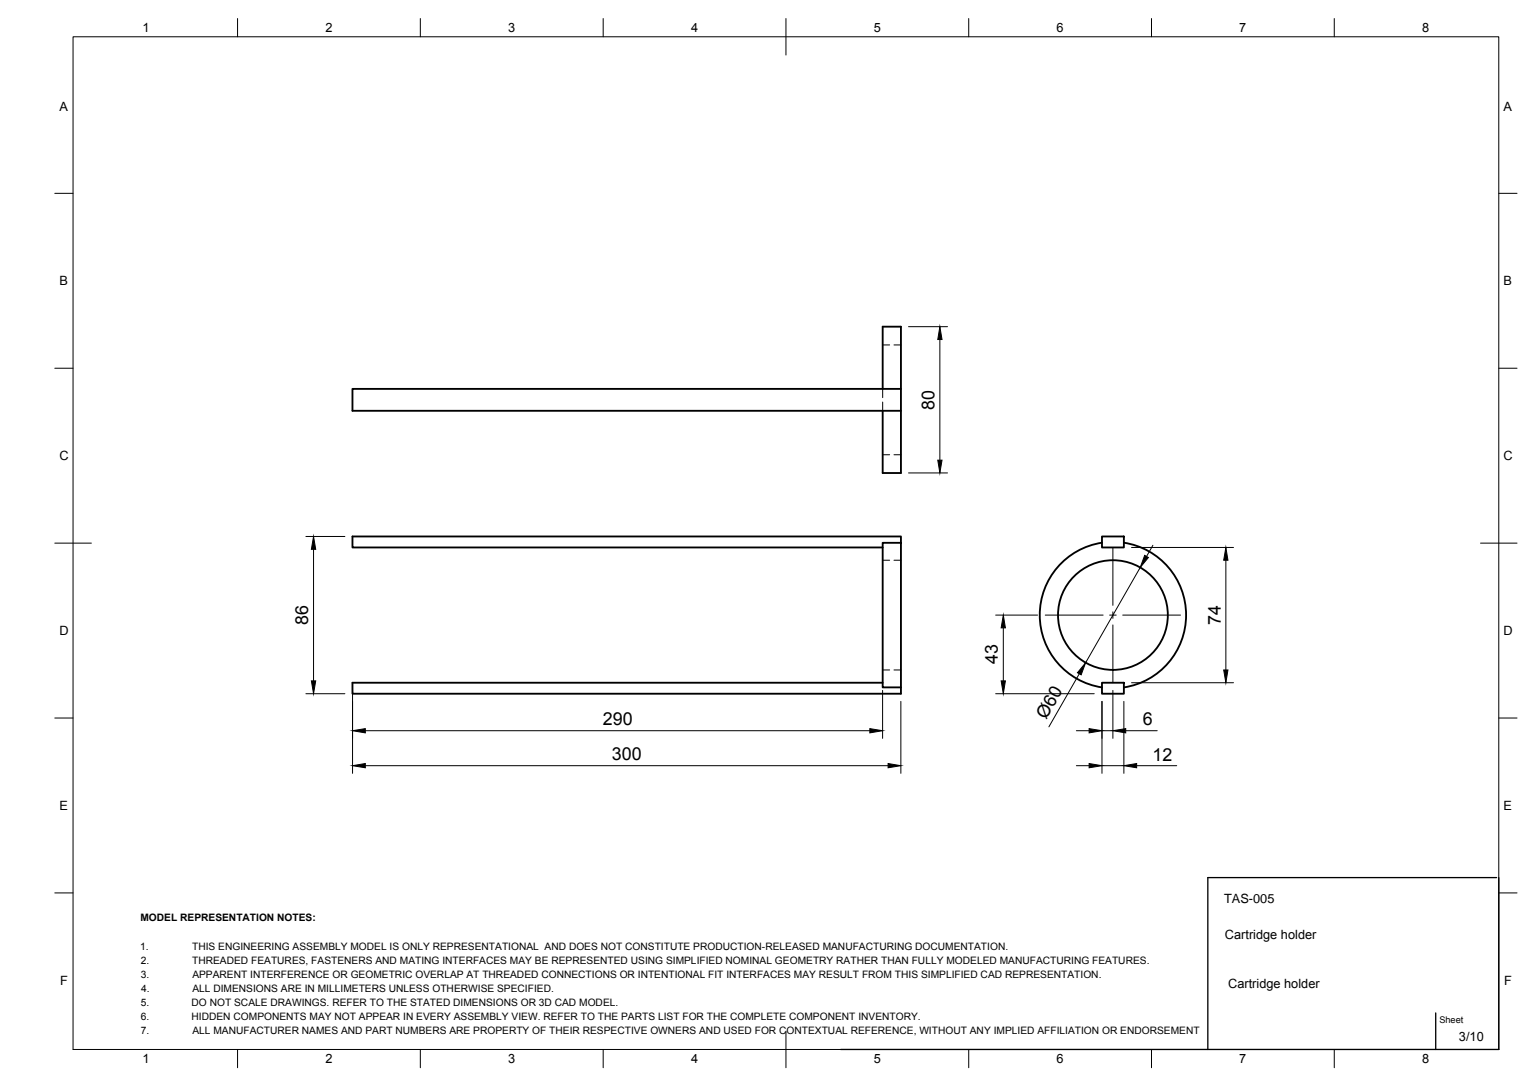
ISO-10303-21;
HEADER;
/* Generated by software containing ST-Developer
 * from STEP Tools, Inc. (www.steptools.com) 
 */

FILE_DESCRIPTION(
/* description */ ('STEP AP214'),
/* implementation_level */ '2;1');

FILE_NAME(
/* name */ 'Cartridge holder.step',
/* time_stamp */ '2026-11-04T19:54:22-08:00',
/* author */ (''),
/* organization */ (''),
/* preprocessor_version */ 'ST-DEVELOPER v20.2',
/* originating_system */ 'Autodesk Translation Framework v15.17.0.0',
/* authorisation */ '');

FILE_SCHEMA (('AUTOMOTIVE_DESIGN { 1 0 10303 214 3 1 1 }'));
ENDSEC;

DATA;
#10=MECHANICAL_DESIGN_GEOMETRIC_PRESENTATION_REPRESENTATION('',(#239),#14084);
#221=SHAPE_REPRESENTATION_RELATIONSHIP('SRR','None',#14120,#230);
#230=ADVANCED_BREP_SHAPE_REPRESENTATION('',(#248),#14075);
#239=STYLED_ITEM('',(#14174),#248);
#248=MANIFOLD_SOLID_BREP('Body1',#3465);
#257=FACE_BOUND('',#558,.T.);
#258=FACE_BOUND('',#561,.T.);
#285=PLANE('',#3582);
#286=PLANE('',#3586);
#287=PLANE('',#3587);
#288=PLANE('',#3588);
#289=PLANE('',#3589);
#290=PLANE('',#3590);
#291=PLANE('',#3591);
#292=PLANE('',#3592);
#293=PLANE('',#3593);
#294=PLANE('',#3594);
#295=PLANE('',#3595);
#296=PLANE('',#3596);
#365=FACE_OUTER_BOUND('',#555,.T.);
#366=FACE_OUTER_BOUND('',#556,.T.);
#367=FACE_OUTER_BOUND('',#557,.T.);
#368=FACE_OUTER_BOUND('',#559,.T.);
#369=FACE_OUTER_BOUND('',#560,.T.);
#370=FACE_OUTER_BOUND('',#562,.T.);
#371=FACE_OUTER_BOUND('',#563,.T.);
#372=FACE_OUTER_BOUND('',#564,.T.);
#373=FACE_OUTER_BOUND('',#565,.T.);
#374=FACE_OUTER_BOUND('',#566,.T.);
#375=FACE_OUTER_BOUND('',#567,.T.);
#376=FACE_OUTER_BOUND('',#568,.T.);
#377=FACE_OUTER_BOUND('',#569,.T.);
#378=FACE_OUTER_BOUND('',#570,.T.);
#379=FACE_OUTER_BOUND('',#571,.T.);
#555=EDGE_LOOP('',(#2197,#2198,#2199,#2200));
#556=EDGE_LOOP('',(#2201,#2202,#2203,#2204));
#557=EDGE_LOOP('',(#2205,#2206,#2207,#2208,#2209,#2210,#2211,#2212));
#558=EDGE_LOOP('',(#2213));
#559=EDGE_LOOP('',(#2214,#2215,#2216,#2217));
#560=EDGE_LOOP('',(#2218,#2219,#2220,#2221,#2222,#2223,#2224,#2225));
#561=EDGE_LOOP('',(#2226));
#562=EDGE_LOOP('',(#2227,#2228,#2229,#2230));
#563=EDGE_LOOP('',(#2231,#2232,#2233,#2234,#2235,#2236));
#564=EDGE_LOOP('',(#2237,#2238,#2239,#2240));
#565=EDGE_LOOP('',(#2241,#2242,#2243,#2244,#2245,#2246));
#566=EDGE_LOOP('',(#2247,#2248,#2249,#2250));
#567=EDGE_LOOP('',(#2251,#2252,#2253,#2254));
#568=EDGE_LOOP('',(#2255,#2256,#2257,#2258,#2259,#2260));
#569=EDGE_LOOP('',(#2261,#2262,#2263,#2264));
#570=EDGE_LOOP('',(#2265,#2266,#2267,#2268,#2269,#2270));
#571=EDGE_LOOP('',(#2271,#2272,#2273,#2274));
#773=LINE('',#4707,#1030);
#774=LINE('',#4714,#1031);
#775=LINE('',#4717,#1032);
#776=LINE('',#4720,#1033);
#777=LINE('',#4722,#1034);
#778=LINE('',#4724,#1035);
#779=LINE('',#4728,#1036);
#780=LINE('',#4730,#1037);
#781=LINE('',#4731,#1038);
#782=LINE('',#4734,#1039);
#783=LINE('',#4737,#1040);
#784=LINE('',#4740,#1041);
#785=LINE('',#4742,#1042);
#786=LINE('',#4743,#1043);
#787=LINE('',#4745,#1044);
#788=LINE('',#4747,#1045);
#789=LINE('',#4748,#1046);
#790=LINE('',#4751,#1047);
#791=LINE('',#4753,#1048);
#792=LINE('',#4754,#1049);
#793=LINE('',#4757,#1050);
#794=LINE('',#4758,#1051);
#795=LINE('',#4761,#1052);
#796=LINE('',#4762,#1053);
#797=LINE('',#4764,#1054);
#798=LINE('',#4768,#1055);
#799=LINE('',#4770,#1056);
#800=LINE('',#4771,#1057);
#801=LINE('',#4774,#1058);
#802=LINE('',#4775,#1059);
#803=LINE('',#4778,#1060);
#804=LINE('',#4779,#1061);
#805=LINE('',#4781,#1062);
#1030=VECTOR('',#3872,30.);
#1031=VECTOR('',#3879,1000.);
#1032=VECTOR('',#3882,1000.);
#1033=VECTOR('',#3885,1000.);
#1034=VECTOR('',#3886,1000.);
#1035=VECTOR('',#3887,1000.);
#1036=VECTOR('',#3890,1000.);
#1037=VECTOR('',#3891,1000.);
#1038=VECTOR('',#3892,1000.);
#1039=VECTOR('',#3895,1000.);
#1040=VECTOR('',#3898,1000.);
#1041=VECTOR('',#3901,1000.);
#1042=VECTOR('',#3902,1000.);
#1043=VECTOR('',#3903,1000.);
#1044=VECTOR('',#3904,1000.);
#1045=VECTOR('',#3905,1000.);
#1046=VECTOR('',#3906,1000.);
#1047=VECTOR('',#3909,1000.);
#1048=VECTOR('',#3910,1000.);
#1049=VECTOR('',#3911,1000.);
#1050=VECTOR('',#3914,1000.);
#1051=VECTOR('',#3915,1000.);
#1052=VECTOR('',#3918,1000.);
#1053=VECTOR('',#3919,1000.);
#1054=VECTOR('',#3922,1000.);
#1055=VECTOR('',#3927,1000.);
#1056=VECTOR('',#3928,1000.);
#1057=VECTOR('',#3929,1000.);
#1058=VECTOR('',#3932,1000.);
#1059=VECTOR('',#3933,1000.);
#1060=VECTOR('',#3936,1000.);
#1061=VECTOR('',#3937,1000.);
#1062=VECTOR('',#3940,1000.);
#1287=CIRCLE('',#3577,30.);
#1288=CIRCLE('',#3578,30.);
#1289=CIRCLE('',#3580,40.);
#1290=CIRCLE('',#3581,40.);
#1291=CIRCLE('',#3583,40.);
#1292=CIRCLE('',#3585,40.);
#1377=VERTEX_POINT('',#4704);
#1378=VERTEX_POINT('',#4706);
#1379=VERTEX_POINT('',#4710);
#1380=VERTEX_POINT('',#4711);
#1381=VERTEX_POINT('',#4713);
#1382=VERTEX_POINT('',#4715);
#1383=VERTEX_POINT('',#4719);
#1384=VERTEX_POINT('',#4721);
#1385=VERTEX_POINT('',#4723);
#1386=VERTEX_POINT('',#4725);
#1387=VERTEX_POINT('',#4727);
#1388=VERTEX_POINT('',#4729);
#1389=VERTEX_POINT('',#4733);
#1390=VERTEX_POINT('',#4735);
#1391=VERTEX_POINT('',#4739);
#1392=VERTEX_POINT('',#4741);
#1393=VERTEX_POINT('',#4744);
#1394=VERTEX_POINT('',#4746);
#1395=VERTEX_POINT('',#4750);
#1396=VERTEX_POINT('',#4752);
#1397=VERTEX_POINT('',#4756);
#1398=VERTEX_POINT('',#4760);
#1399=VERTEX_POINT('',#4767);
#1400=VERTEX_POINT('',#4769);
#1401=VERTEX_POINT('',#4773);
#1402=VERTEX_POINT('',#4777);
#1702=EDGE_CURVE('',#1377,#1377,#1287,.T.);
#1703=EDGE_CURVE('',#1377,#1378,#773,.T.);
#1704=EDGE_CURVE('',#1378,#1378,#1288,.T.);
#1705=EDGE_CURVE('',#1379,#1380,#1289,.T.);
#1706=EDGE_CURVE('',#1381,#1379,#774,.T.);
#1707=EDGE_CURVE('',#1381,#1382,#1290,.T.);
#1708=EDGE_CURVE('',#1380,#1382,#775,.T.);
#1709=EDGE_CURVE('',#1380,#1383,#776,.T.);
#1710=EDGE_CURVE('',#1383,#1384,#777,.T.);
#1711=EDGE_CURVE('',#1384,#1385,#778,.T.);
#1712=EDGE_CURVE('',#1385,#1386,#1291,.T.);
#1713=EDGE_CURVE('',#1386,#1387,#779,.T.);
#1714=EDGE_CURVE('',#1387,#1388,#780,.T.);
#1715=EDGE_CURVE('',#1388,#1379,#781,.T.);
#1716=EDGE_CURVE('',#1389,#1385,#782,.T.);
#1717=EDGE_CURVE('',#1389,#1390,#1292,.T.);
#1718=EDGE_CURVE('',#1386,#1390,#783,.T.);
#1719=EDGE_CURVE('',#1391,#1389,#784,.T.);
#1720=EDGE_CURVE('',#1392,#1391,#785,.T.);
#1721=EDGE_CURVE('',#1382,#1392,#786,.T.);
#1722=EDGE_CURVE('',#1393,#1381,#787,.T.);
#1723=EDGE_CURVE('',#1394,#1393,#788,.T.);
#1724=EDGE_CURVE('',#1390,#1394,#789,.T.);
#1725=EDGE_CURVE('',#1395,#1393,#790,.T.);
#1726=EDGE_CURVE('',#1396,#1395,#791,.T.);
#1727=EDGE_CURVE('',#1396,#1394,#792,.T.);
#1728=EDGE_CURVE('',#1397,#1388,#793,.T.);
#1729=EDGE_CURVE('',#1395,#1397,#794,.T.);
#1730=EDGE_CURVE('',#1398,#1387,#795,.T.);
#1731=EDGE_CURVE('',#1397,#1398,#796,.T.);
#1732=EDGE_CURVE('',#1398,#1396,#797,.T.);
#1733=EDGE_CURVE('',#1399,#1383,#798,.T.);
#1734=EDGE_CURVE('',#1400,#1399,#799,.T.);
#1735=EDGE_CURVE('',#1400,#1384,#800,.T.);
#1736=EDGE_CURVE('',#1401,#1392,#801,.T.);
#1737=EDGE_CURVE('',#1399,#1401,#802,.T.);
#1738=EDGE_CURVE('',#1402,#1391,#803,.T.);
#1739=EDGE_CURVE('',#1401,#1402,#804,.T.);
#1740=EDGE_CURVE('',#1402,#1400,#805,.T.);
#2197=ORIENTED_EDGE('',*,*,#1702,.T.);
#2198=ORIENTED_EDGE('',*,*,#1703,.T.);
#2199=ORIENTED_EDGE('',*,*,#1704,.F.);
#2200=ORIENTED_EDGE('',*,*,#1703,.F.);
#2201=ORIENTED_EDGE('',*,*,#1705,.F.);
#2202=ORIENTED_EDGE('',*,*,#1706,.F.);
#2203=ORIENTED_EDGE('',*,*,#1707,.T.);
#2204=ORIENTED_EDGE('',*,*,#1708,.F.);
#2205=ORIENTED_EDGE('',*,*,#1705,.T.);
#2206=ORIENTED_EDGE('',*,*,#1709,.T.);
#2207=ORIENTED_EDGE('',*,*,#1710,.T.);
#2208=ORIENTED_EDGE('',*,*,#1711,.T.);
#2209=ORIENTED_EDGE('',*,*,#1712,.T.);
#2210=ORIENTED_EDGE('',*,*,#1713,.T.);
#2211=ORIENTED_EDGE('',*,*,#1714,.T.);
#2212=ORIENTED_EDGE('',*,*,#1715,.T.);
#2213=ORIENTED_EDGE('',*,*,#1702,.F.);
#2214=ORIENTED_EDGE('',*,*,#1716,.F.);
#2215=ORIENTED_EDGE('',*,*,#1717,.T.);
#2216=ORIENTED_EDGE('',*,*,#1718,.F.);
#2217=ORIENTED_EDGE('',*,*,#1712,.F.);
#2218=ORIENTED_EDGE('',*,*,#1717,.F.);
#2219=ORIENTED_EDGE('',*,*,#1719,.F.);
#2220=ORIENTED_EDGE('',*,*,#1720,.F.);
#2221=ORIENTED_EDGE('',*,*,#1721,.F.);
#2222=ORIENTED_EDGE('',*,*,#1707,.F.);
#2223=ORIENTED_EDGE('',*,*,#1722,.F.);
#2224=ORIENTED_EDGE('',*,*,#1723,.F.);
#2225=ORIENTED_EDGE('',*,*,#1724,.F.);
#2226=ORIENTED_EDGE('',*,*,#1704,.T.);
#2227=ORIENTED_EDGE('',*,*,#1723,.T.);
#2228=ORIENTED_EDGE('',*,*,#1725,.F.);
#2229=ORIENTED_EDGE('',*,*,#1726,.F.);
#2230=ORIENTED_EDGE('',*,*,#1727,.T.);
#2231=ORIENTED_EDGE('',*,*,#1715,.F.);
#2232=ORIENTED_EDGE('',*,*,#1728,.F.);
#2233=ORIENTED_EDGE('',*,*,#1729,.F.);
#2234=ORIENTED_EDGE('',*,*,#1725,.T.);
#2235=ORIENTED_EDGE('',*,*,#1722,.T.);
#2236=ORIENTED_EDGE('',*,*,#1706,.T.);
#2237=ORIENTED_EDGE('',*,*,#1714,.F.);
#2238=ORIENTED_EDGE('',*,*,#1730,.F.);
#2239=ORIENTED_EDGE('',*,*,#1731,.F.);
#2240=ORIENTED_EDGE('',*,*,#1728,.T.);
#2241=ORIENTED_EDGE('',*,*,#1713,.F.);
#2242=ORIENTED_EDGE('',*,*,#1718,.T.);
#2243=ORIENTED_EDGE('',*,*,#1724,.T.);
#2244=ORIENTED_EDGE('',*,*,#1727,.F.);
#2245=ORIENTED_EDGE('',*,*,#1732,.F.);
#2246=ORIENTED_EDGE('',*,*,#1730,.T.);
#2247=ORIENTED_EDGE('',*,*,#1726,.T.);
#2248=ORIENTED_EDGE('',*,*,#1729,.T.);
#2249=ORIENTED_EDGE('',*,*,#1731,.T.);
#2250=ORIENTED_EDGE('',*,*,#1732,.T.);
#2251=ORIENTED_EDGE('',*,*,#1710,.F.);
#2252=ORIENTED_EDGE('',*,*,#1733,.F.);
#2253=ORIENTED_EDGE('',*,*,#1734,.F.);
#2254=ORIENTED_EDGE('',*,*,#1735,.T.);
#2255=ORIENTED_EDGE('',*,*,#1709,.F.);
#2256=ORIENTED_EDGE('',*,*,#1708,.T.);
#2257=ORIENTED_EDGE('',*,*,#1721,.T.);
#2258=ORIENTED_EDGE('',*,*,#1736,.F.);
#2259=ORIENTED_EDGE('',*,*,#1737,.F.);
#2260=ORIENTED_EDGE('',*,*,#1733,.T.);
#2261=ORIENTED_EDGE('',*,*,#1720,.T.);
#2262=ORIENTED_EDGE('',*,*,#1738,.F.);
#2263=ORIENTED_EDGE('',*,*,#1739,.F.);
#2264=ORIENTED_EDGE('',*,*,#1736,.T.);
#2265=ORIENTED_EDGE('',*,*,#1711,.F.);
#2266=ORIENTED_EDGE('',*,*,#1735,.F.);
#2267=ORIENTED_EDGE('',*,*,#1740,.F.);
#2268=ORIENTED_EDGE('',*,*,#1738,.T.);
#2269=ORIENTED_EDGE('',*,*,#1719,.T.);
#2270=ORIENTED_EDGE('',*,*,#1716,.T.);
#2271=ORIENTED_EDGE('',*,*,#1734,.T.);
#2272=ORIENTED_EDGE('',*,*,#1737,.T.);
#2273=ORIENTED_EDGE('',*,*,#1739,.T.);
#2274=ORIENTED_EDGE('',*,*,#1740,.T.);
#3187=CYLINDRICAL_SURFACE('',#3576,30.);
#3188=CYLINDRICAL_SURFACE('',#3579,40.);
#3189=CYLINDRICAL_SURFACE('',#3584,40.);
#3275=ADVANCED_FACE('',(#365),#3187,.F.);
#3276=ADVANCED_FACE('',(#366),#3188,.T.);
#3277=ADVANCED_FACE('',(#367,#257),#285,.T.);
#3278=ADVANCED_FACE('',(#368),#3189,.T.);
#3279=ADVANCED_FACE('',(#369,#258),#286,.F.);
#3280=ADVANCED_FACE('',(#370),#287,.F.);
#3281=ADVANCED_FACE('',(#371),#288,.F.);
#3282=ADVANCED_FACE('',(#372),#289,.F.);
#3283=ADVANCED_FACE('',(#373),#290,.F.);
#3284=ADVANCED_FACE('',(#374),#291,.T.);
#3285=ADVANCED_FACE('',(#375),#292,.F.);
#3286=ADVANCED_FACE('',(#376),#293,.F.);
#3287=ADVANCED_FACE('',(#377),#294,.F.);
#3288=ADVANCED_FACE('',(#378),#295,.F.);
#3289=ADVANCED_FACE('',(#379),#296,.F.);
#3465=CLOSED_SHELL('',(#3275,#3276,#3277,#3278,#3279,#3280,#3281,#3282,
#3283,#3284,#3285,#3286,#3287,#3288,#3289));
#3575=AXIS2_PLACEMENT_3D('',#4702,#3866,#3867);
#3576=AXIS2_PLACEMENT_3D('',#4703,#3868,#3869);
#3577=AXIS2_PLACEMENT_3D('',#4705,#3870,#3871);
#3578=AXIS2_PLACEMENT_3D('',#4708,#3873,#3874);
#3579=AXIS2_PLACEMENT_3D('',#4709,#3875,#3876);
#3580=AXIS2_PLACEMENT_3D('',#4712,#3877,#3878);
#3581=AXIS2_PLACEMENT_3D('',#4716,#3880,#3881);
#3582=AXIS2_PLACEMENT_3D('',#4718,#3883,#3884);
#3583=AXIS2_PLACEMENT_3D('',#4726,#3888,#3889);
#3584=AXIS2_PLACEMENT_3D('',#4732,#3893,#3894);
#3585=AXIS2_PLACEMENT_3D('',#4736,#3896,#3897);
#3586=AXIS2_PLACEMENT_3D('',#4738,#3899,#3900);
#3587=AXIS2_PLACEMENT_3D('',#4749,#3907,#3908);
#3588=AXIS2_PLACEMENT_3D('',#4755,#3912,#3913);
#3589=AXIS2_PLACEMENT_3D('',#4759,#3916,#3917);
#3590=AXIS2_PLACEMENT_3D('',#4763,#3920,#3921);
#3591=AXIS2_PLACEMENT_3D('',#4765,#3923,#3924);
#3592=AXIS2_PLACEMENT_3D('',#4766,#3925,#3926);
#3593=AXIS2_PLACEMENT_3D('',#4772,#3930,#3931);
#3594=AXIS2_PLACEMENT_3D('',#4776,#3934,#3935);
#3595=AXIS2_PLACEMENT_3D('',#4780,#3938,#3939);
#3596=AXIS2_PLACEMENT_3D('',#4782,#3941,#3942);
#3866=DIRECTION('axis',(0.,0.,1.));
#3867=DIRECTION('refdir',(1.,0.,0.));
#3868=DIRECTION('center_axis',(0.,-1.,0.));
#3869=DIRECTION('ref_axis',(0.,0.,-1.));
#3870=DIRECTION('center_axis',(0.,1.,0.));
#3871=DIRECTION('ref_axis',(0.,0.,1.));
#3872=DIRECTION('',(0.,-1.,0.));
#3873=DIRECTION('center_axis',(0.,1.,0.));
#3874=DIRECTION('ref_axis',(0.,0.,1.));
#3875=DIRECTION('center_axis',(0.,-1.,0.));
#3876=DIRECTION('ref_axis',(0.,0.,-1.));
#3877=DIRECTION('center_axis',(0.,1.,0.));
#3878=DIRECTION('ref_axis',(1.,0.,0.));
#3879=DIRECTION('',(0.,1.,0.));
#3880=DIRECTION('center_axis',(0.,1.,0.));
#3881=DIRECTION('ref_axis',(1.,0.,0.));
#3882=DIRECTION('',(0.,-1.,0.));
#3883=DIRECTION('center_axis',(0.,1.,0.));
#3884=DIRECTION('ref_axis',(0.,0.,1.));
#3885=DIRECTION('',(1.,0.,0.));
#3886=DIRECTION('',(0.,0.,1.));
#3887=DIRECTION('',(-1.,0.,0.));
#3888=DIRECTION('center_axis',(0.,1.,0.));
#3889=DIRECTION('ref_axis',(1.,0.,0.));
#3890=DIRECTION('',(-1.,0.,2.89120579329468E-16));
#3891=DIRECTION('',(0.,0.,-1.));
#3892=DIRECTION('',(1.,0.,-2.89120579329468E-16));
#3893=DIRECTION('center_axis',(0.,-1.,0.));
#3894=DIRECTION('ref_axis',(-1.22464679914735E-16,0.,1.));
#3895=DIRECTION('',(0.,1.,0.));
#3896=DIRECTION('center_axis',(0.,1.,0.));
#3897=DIRECTION('ref_axis',(1.,0.,0.));
#3898=DIRECTION('',(0.,-1.,0.));
#3899=DIRECTION('center_axis',(0.,1.,0.));
#3900=DIRECTION('ref_axis',(0.,0.,1.));
#3901=DIRECTION('',(1.,0.,0.));
#3902=DIRECTION('',(0.,0.,1.));
#3903=DIRECTION('',(-1.,0.,0.));
#3904=DIRECTION('',(-1.,0.,2.89120579329468E-16));
#3905=DIRECTION('',(0.,0.,-1.));
#3906=DIRECTION('',(1.,0.,-2.89120579329468E-16));
#3907=DIRECTION('center_axis',(-1.,0.,0.));
#3908=DIRECTION('ref_axis',(0.,0.,1.));
#3909=DIRECTION('',(0.,-1.,0.));
#3910=DIRECTION('',(0.,0.,-1.));
#3911=DIRECTION('',(0.,-1.,0.));
#3912=DIRECTION('center_axis',(2.89120579329468E-16,0.,1.));
#3913=DIRECTION('ref_axis',(1.,0.,-2.89120579329468E-16));
#3914=DIRECTION('',(0.,-1.,0.));
#3915=DIRECTION('',(-1.,0.,2.89120579329468E-16));
#3916=DIRECTION('center_axis',(1.,0.,0.));
#3917=DIRECTION('ref_axis',(0.,0.,-1.));
#3918=DIRECTION('',(0.,-1.,0.));
#3919=DIRECTION('',(0.,0.,1.));
#3920=DIRECTION('center_axis',(-2.89120579329468E-16,0.,-1.));
#3921=DIRECTION('ref_axis',(-1.,0.,2.89120579329468E-16));
#3922=DIRECTION('',(1.,0.,-2.89120579329468E-16));
#3923=DIRECTION('center_axis',(0.,1.,0.));
#3924=DIRECTION('ref_axis',(0.,0.,1.));
#3925=DIRECTION('center_axis',(-1.,0.,0.));
#3926=DIRECTION('ref_axis',(0.,0.,1.));
#3927=DIRECTION('',(0.,-1.,0.));
#3928=DIRECTION('',(0.,0.,-1.));
#3929=DIRECTION('',(0.,-1.,0.));
#3930=DIRECTION('center_axis',(0.,0.,1.));
#3931=DIRECTION('ref_axis',(1.,0.,0.));
#3932=DIRECTION('',(0.,-1.,0.));
#3933=DIRECTION('',(-1.,0.,0.));
#3934=DIRECTION('center_axis',(1.,0.,0.));
#3935=DIRECTION('ref_axis',(0.,0.,-1.));
#3936=DIRECTION('',(0.,-1.,0.));
#3937=DIRECTION('',(0.,0.,1.));
#3938=DIRECTION('center_axis',(0.,0.,-1.));
#3939=DIRECTION('ref_axis',(-1.,0.,0.));
#3940=DIRECTION('',(1.,0.,0.));
#3941=DIRECTION('center_axis',(0.,-1.,0.));
#3942=DIRECTION('ref_axis',(0.,0.,-1.));
#4702=CARTESIAN_POINT('',(0.,0.,0.));
#4703=CARTESIAN_POINT('Origin',(0.,10.,0.));
#4704=CARTESIAN_POINT('',(-3.67394039744206E-15,10.,30.));
#4705=CARTESIAN_POINT('Origin',(0.,10.,0.));
#4706=CARTESIAN_POINT('',(-3.67394039744206E-15,1.11022302462516E-15,30.));
#4707=CARTESIAN_POINT('',(-3.67394039744206E-15,10.,30.));
#4708=CARTESIAN_POINT('Origin',(0.,0.,0.));
#4709=CARTESIAN_POINT('Origin',(0.,10.,0.));
#4710=CARTESIAN_POINT('',(39.5474398665704,10.,-6.));
#4711=CARTESIAN_POINT('',(-39.5474398665704,10.,-5.99999999999999));
#4712=CARTESIAN_POINT('Origin',(0.,10.,0.));
#4713=CARTESIAN_POINT('',(39.5474398665704,0.,-6.));
#4714=CARTESIAN_POINT('',(39.5474398665704,10.,-6.));
#4715=CARTESIAN_POINT('',(-39.5474398665704,0.,-5.99999999999999));
#4716=CARTESIAN_POINT('Origin',(0.,0.,0.));
#4717=CARTESIAN_POINT('',(-39.5474398665704,10.,-5.99999999999999));
#4718=CARTESIAN_POINT('Origin',(0.,10.,0.));
#4719=CARTESIAN_POINT('',(-37.,10.,-5.99999999999999));
#4720=CARTESIAN_POINT('',(0.,10.,-5.99999999999999));
#4721=CARTESIAN_POINT('',(-37.,10.,6.00000000000001));
#4722=CARTESIAN_POINT('',(-37.,10.,0.));
#4723=CARTESIAN_POINT('',(-39.5474398665704,10.,6.00000000000001));
#4724=CARTESIAN_POINT('',(0.,10.,6.00000000000001));
#4725=CARTESIAN_POINT('',(39.5474398665704,10.,6.));
#4726=CARTESIAN_POINT('Origin',(0.,10.,0.));
#4727=CARTESIAN_POINT('',(37.,10.,6.00000000000001));
#4728=CARTESIAN_POINT('',(1.73472347597681E-15,10.,6.00000000000002));
#4729=CARTESIAN_POINT('',(37.,10.,-6.));
#4730=CARTESIAN_POINT('',(37.,10.,0.));
#4731=CARTESIAN_POINT('',(-1.7347234759768E-15,10.,-5.99999999999999));
#4732=CARTESIAN_POINT('Origin',(0.,10.,0.));
#4733=CARTESIAN_POINT('',(-39.5474398665704,0.,6.00000000000001));
#4734=CARTESIAN_POINT('',(-39.5474398665704,10.,6.00000000000001));
#4735=CARTESIAN_POINT('',(39.5474398665704,0.,6.));
#4736=CARTESIAN_POINT('Origin',(0.,0.,0.));
#4737=CARTESIAN_POINT('',(39.5474398665704,10.,6.));
#4738=CARTESIAN_POINT('Origin',(0.,0.,0.));
#4739=CARTESIAN_POINT('',(-43.,0.,6.00000000000001));
#4740=CARTESIAN_POINT('',(-43.,0.,6.00000000000001));
#4741=CARTESIAN_POINT('',(-43.,0.,-5.99999999999999));
#4742=CARTESIAN_POINT('',(-43.,0.,6.00000000000001));
#4743=CARTESIAN_POINT('',(-43.,0.,-5.99999999999999));
#4744=CARTESIAN_POINT('',(43.,0.,-6.));
#4745=CARTESIAN_POINT('',(43.,0.,-6.));
#4746=CARTESIAN_POINT('',(43.,0.,6.));
#4747=CARTESIAN_POINT('',(43.,0.,6.));
#4748=CARTESIAN_POINT('',(43.,0.,6.));
#4749=CARTESIAN_POINT('Origin',(43.,300.,6.));
#4750=CARTESIAN_POINT('',(43.,300.,-6.));
#4751=CARTESIAN_POINT('',(43.,300.,-6.));
#4752=CARTESIAN_POINT('',(43.,300.,6.));
#4753=CARTESIAN_POINT('',(43.,300.,6.));
#4754=CARTESIAN_POINT('',(43.,300.,6.));
#4755=CARTESIAN_POINT('Origin',(43.,300.,-6.));
#4756=CARTESIAN_POINT('',(37.,300.,-6.));
#4757=CARTESIAN_POINT('',(37.,300.,-6.));
#4758=CARTESIAN_POINT('',(43.,300.,-6.));
#4759=CARTESIAN_POINT('Origin',(37.,300.,6.00000000000001));
#4760=CARTESIAN_POINT('',(37.,300.,6.00000000000001));
#4761=CARTESIAN_POINT('',(37.,300.,6.00000000000001));
#4762=CARTESIAN_POINT('',(37.,300.,6.00000000000001));
#4763=CARTESIAN_POINT('Origin',(43.,300.,6.));
#4764=CARTESIAN_POINT('',(43.,300.,6.));
#4765=CARTESIAN_POINT('Origin',(0.,300.,0.));
#4766=CARTESIAN_POINT('Origin',(-37.,300.,6.00000000000001));
#4767=CARTESIAN_POINT('',(-37.,300.,-5.99999999999999));
#4768=CARTESIAN_POINT('',(-37.,300.,-5.99999999999999));
#4769=CARTESIAN_POINT('',(-37.,300.,6.00000000000001));
#4770=CARTESIAN_POINT('',(-37.,300.,6.00000000000001));
#4771=CARTESIAN_POINT('',(-37.,300.,6.00000000000001));
#4772=CARTESIAN_POINT('Origin',(-43.,300.,-5.99999999999999));
#4773=CARTESIAN_POINT('',(-43.,300.,-5.99999999999999));
#4774=CARTESIAN_POINT('',(-43.,300.,-5.99999999999999));
#4775=CARTESIAN_POINT('',(-43.,300.,-5.99999999999999));
#4776=CARTESIAN_POINT('Origin',(-43.,300.,6.00000000000001));
#4777=CARTESIAN_POINT('',(-43.,300.,6.00000000000001));
#4778=CARTESIAN_POINT('',(-43.,300.,6.00000000000001));
#4779=CARTESIAN_POINT('',(-43.,300.,6.00000000000001));
#4780=CARTESIAN_POINT('Origin',(-43.,300.,6.00000000000001));
#4781=CARTESIAN_POINT('',(-43.,300.,6.00000000000001));
#4782=CARTESIAN_POINT('Origin',(0.,300.,0.));
#14064=UNCERTAINTY_MEASURE_WITH_UNIT(LENGTH_MEASURE(0.01),#14085,
'DISTANCE_ACCURACY_VALUE',
'Maximum model space distance between geometric entities at asserted c
onnectivities');
#14073=UNCERTAINTY_MEASURE_WITH_UNIT(LENGTH_MEASURE(0.01),#14085,
'DISTANCE_ACCURACY_VALUE',
'Maximum model space distance between geometric entities at asserted c
onnectivities');
#14075=(
GEOMETRIC_REPRESENTATION_CONTEXT(3)
GLOBAL_UNCERTAINTY_ASSIGNED_CONTEXT((#14064))
GLOBAL_UNIT_ASSIGNED_CONTEXT((#14085,#14087,#14088))
REPRESENTATION_CONTEXT('','3D')
);
#14084=(
GEOMETRIC_REPRESENTATION_CONTEXT(3)
GLOBAL_UNCERTAINTY_ASSIGNED_CONTEXT((#14073))
GLOBAL_UNIT_ASSIGNED_CONTEXT((#14085,#14087,#14088))
REPRESENTATION_CONTEXT('','3D')
);
#14085=(
LENGTH_UNIT()
NAMED_UNIT(*)
SI_UNIT(.MILLI.,.METRE.)
);
#14087=(
NAMED_UNIT(*)
PLANE_ANGLE_UNIT()
SI_UNIT($,.RADIAN.)
);
#14088=(
NAMED_UNIT(*)
SI_UNIT($,.STERADIAN.)
SOLID_ANGLE_UNIT()
);
#14090=SHAPE_DEFINITION_REPRESENTATION(#14100,#14120);
#14100=PRODUCT_DEFINITION_SHAPE('',$,#14131);
#14120=SHAPE_REPRESENTATION('',(#3575),#14075);
#14129=PRODUCT_DEFINITION_CONTEXT('part definition',#14161,'design');
#14131=PRODUCT_DEFINITION('Cartridge holder','Cartridge holder',#14141,
#14129);
#14141=PRODUCT_DEFINITION_FORMATION('',$,#14164);
#14161=APPLICATION_CONTEXT(
'Core Data for Automotive Mechanical Design Process');
#14162=PRODUCT_CONTEXT('part definition',#14161,'mechanical');
#14164=PRODUCT('Cartridge holder','Cartridge holder',$,(#14162));
#14174=PRESENTATION_STYLE_ASSIGNMENT((#14180));
#14180=SURFACE_STYLE_USAGE(.BOTH.,#14186);
#14186=SURFACE_SIDE_STYLE('',(#14192));
#14192=SURFACE_STYLE_FILL_AREA(#14198);
#14198=FILL_AREA_STYLE('Opaque(97,158,199)',(#14204));
#14204=FILL_AREA_STYLE_COLOUR('Opaque(97,158,199)',#14210);
#14210=COLOUR_RGB('Opaque(97,158,199)',0.380392156862745,0.619607843137255,
0.780392156862745);
ENDSEC;
END-ISO-10303-21;
